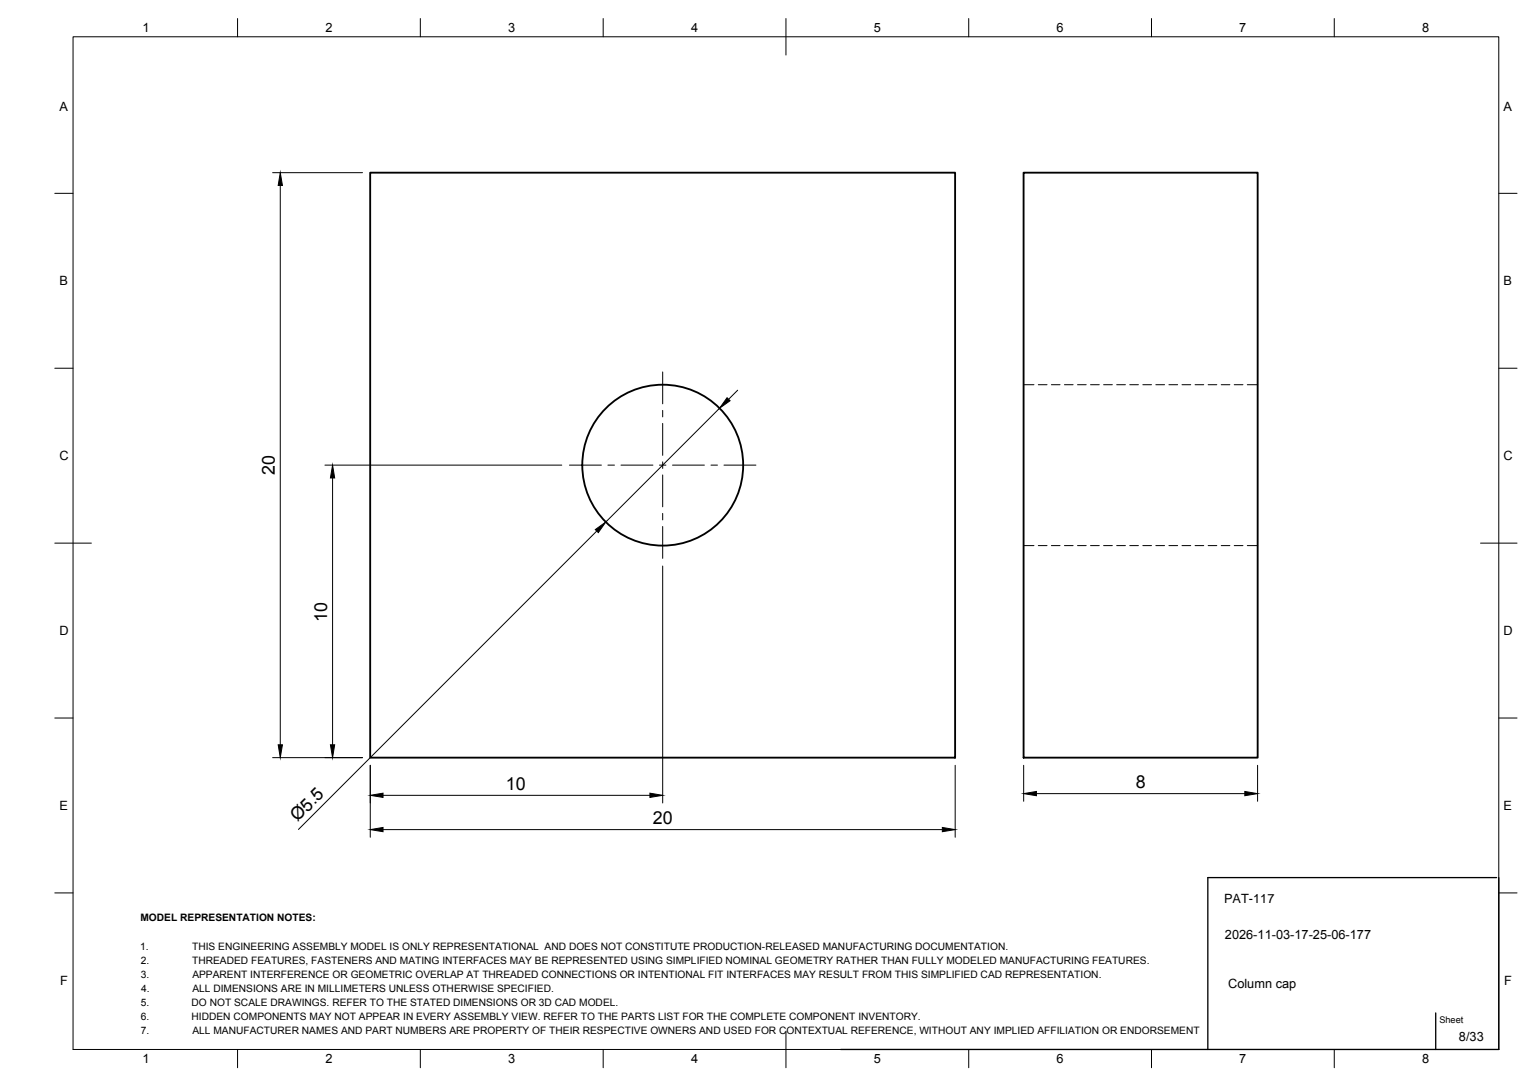
ISO-10303-21;
HEADER;
/* Generated by software containing ST-Developer
 * from STEP Tools, Inc. (www.steptools.com) 
 */

FILE_DESCRIPTION(
/* description */ ('Counterbalanced vertical column'),
/* implementation_level */ '2;1');

FILE_NAME(
/* name */ 'Column cap.step',
/* time_stamp */ '2026-10-29T16:47:22-07:00',
/* author */ (''),
/* organization */ (''),
/* preprocessor_version */ 'ST-DEVELOPER v20.2',
/* originating_system */ 'Autodesk Translation Framework v15.17.0.0',
/* authorisation */ '');

FILE_SCHEMA (('AUTOMOTIVE_DESIGN { 1 0 10303 214 3 1 1 }'));
ENDSEC;

DATA;
#10=MECHANICAL_DESIGN_GEOMETRIC_PRESENTATION_REPRESENTATION('',(#353),#15040);
#283=SHAPE_REPRESENTATION_RELATIONSHIP('SRR','None',#15187,#318);
#318=ADVANCED_BREP_SHAPE_REPRESENTATION('',(#388),#15006);
#353=STYLED_ITEM('',(#15471),#388);
#388=MANIFOLD_SOLID_BREP('Body1',#7076);
#422=FACE_BOUND('',#1270,.T.);
#423=FACE_BOUND('',#1272,.T.);
#553=PLANE('',#7544);
#554=PLANE('',#7545);
#555=PLANE('',#7546);
#556=PLANE('',#7547);
#557=PLANE('',#7548);
#558=PLANE('',#7549);
#853=FACE_OUTER_BOUND('',#1264,.T.);
#854=FACE_OUTER_BOUND('',#1265,.T.);
#855=FACE_OUTER_BOUND('',#1266,.T.);
#856=FACE_OUTER_BOUND('',#1267,.T.);
#857=FACE_OUTER_BOUND('',#1268,.T.);
#858=FACE_OUTER_BOUND('',#1269,.T.);
#859=FACE_OUTER_BOUND('',#1271,.T.);
#1264=EDGE_LOOP('',(#4890,#4891,#4892,#4893));
#1265=EDGE_LOOP('',(#4894,#4895,#4896,#4897));
#1266=EDGE_LOOP('',(#4898,#4899,#4900,#4901));
#1267=EDGE_LOOP('',(#4902,#4903,#4904,#4905));
#1268=EDGE_LOOP('',(#4906,#4907,#4908,#4909));
#1269=EDGE_LOOP('',(#4910,#4911,#4912,#4913));
#1270=EDGE_LOOP('',(#4914));
#1271=EDGE_LOOP('',(#4915,#4916,#4917,#4918));
#1272=EDGE_LOOP('',(#4919));
#1792=LINE('',#10460,#2463);
#1793=LINE('',#10465,#2464);
#1794=LINE('',#10467,#2465);
#1795=LINE('',#10469,#2466);
#1796=LINE('',#10470,#2467);
#1797=LINE('',#10473,#2468);
#1798=LINE('',#10475,#2469);
#1799=LINE('',#10476,#2470);
#1800=LINE('',#10479,#2471);
#1801=LINE('',#10481,#2472);
#1802=LINE('',#10482,#2473);
#1803=LINE('',#10484,#2474);
#1804=LINE('',#10485,#2475);
#2463=VECTOR('',#8352,0.275);
#2464=VECTOR('',#8357,1.);
#2465=VECTOR('',#8358,1.);
#2466=VECTOR('',#8359,1.);
#2467=VECTOR('',#8360,1.);
#2468=VECTOR('',#8363,1.);
#2469=VECTOR('',#8364,1.);
#2470=VECTOR('',#8365,1.);
#2471=VECTOR('',#8368,1.);
#2472=VECTOR('',#8369,1.);
#2473=VECTOR('',#8370,1.);
#2474=VECTOR('',#8373,1.);
#2475=VECTOR('',#8374,1.);
#3103=CIRCLE('',#7542,0.275);
#3104=CIRCLE('',#7543,0.275);
#3340=VERTEX_POINT('',#10457);
#3341=VERTEX_POINT('',#10459);
#3342=VERTEX_POINT('',#10463);
#3343=VERTEX_POINT('',#10464);
#3344=VERTEX_POINT('',#10466);
#3345=VERTEX_POINT('',#10468);
#3346=VERTEX_POINT('',#10472);
#3347=VERTEX_POINT('',#10474);
#3348=VERTEX_POINT('',#10478);
#3349=VERTEX_POINT('',#10480);
#3946=EDGE_CURVE('',#3340,#3340,#3103,.T.);
#3947=EDGE_CURVE('',#3340,#3341,#1792,.T.);
#3948=EDGE_CURVE('',#3341,#3341,#3104,.T.);
#3949=EDGE_CURVE('',#3342,#3343,#1793,.T.);
#3950=EDGE_CURVE('',#3343,#3344,#1794,.T.);
#3951=EDGE_CURVE('',#3345,#3344,#1795,.T.);
#3952=EDGE_CURVE('',#3342,#3345,#1796,.T.);
#3953=EDGE_CURVE('',#3346,#3342,#1797,.T.);
#3954=EDGE_CURVE('',#3347,#3345,#1798,.T.);
#3955=EDGE_CURVE('',#3346,#3347,#1799,.T.);
#3956=EDGE_CURVE('',#3348,#3346,#1800,.T.);
#3957=EDGE_CURVE('',#3349,#3347,#1801,.T.);
#3958=EDGE_CURVE('',#3348,#3349,#1802,.T.);
#3959=EDGE_CURVE('',#3343,#3348,#1803,.T.);
#3960=EDGE_CURVE('',#3344,#3349,#1804,.T.);
#4890=ORIENTED_EDGE('',*,*,#3946,.F.);
#4891=ORIENTED_EDGE('',*,*,#3947,.T.);
#4892=ORIENTED_EDGE('',*,*,#3948,.F.);
#4893=ORIENTED_EDGE('',*,*,#3947,.F.);
#4894=ORIENTED_EDGE('',*,*,#3949,.T.);
#4895=ORIENTED_EDGE('',*,*,#3950,.T.);
#4896=ORIENTED_EDGE('',*,*,#3951,.F.);
#4897=ORIENTED_EDGE('',*,*,#3952,.F.);
#4898=ORIENTED_EDGE('',*,*,#3953,.T.);
#4899=ORIENTED_EDGE('',*,*,#3952,.T.);
#4900=ORIENTED_EDGE('',*,*,#3954,.F.);
#4901=ORIENTED_EDGE('',*,*,#3955,.F.);
#4902=ORIENTED_EDGE('',*,*,#3956,.T.);
#4903=ORIENTED_EDGE('',*,*,#3955,.T.);
#4904=ORIENTED_EDGE('',*,*,#3957,.F.);
#4905=ORIENTED_EDGE('',*,*,#3958,.F.);
#4906=ORIENTED_EDGE('',*,*,#3959,.T.);
#4907=ORIENTED_EDGE('',*,*,#3958,.T.);
#4908=ORIENTED_EDGE('',*,*,#3960,.F.);
#4909=ORIENTED_EDGE('',*,*,#3950,.F.);
#4910=ORIENTED_EDGE('',*,*,#3960,.T.);
#4911=ORIENTED_EDGE('',*,*,#3957,.T.);
#4912=ORIENTED_EDGE('',*,*,#3954,.T.);
#4913=ORIENTED_EDGE('',*,*,#3951,.T.);
#4914=ORIENTED_EDGE('',*,*,#3948,.T.);
#4915=ORIENTED_EDGE('',*,*,#3959,.F.);
#4916=ORIENTED_EDGE('',*,*,#3949,.F.);
#4917=ORIENTED_EDGE('',*,*,#3953,.F.);
#4918=ORIENTED_EDGE('',*,*,#3956,.F.);
#4919=ORIENTED_EDGE('',*,*,#3946,.T.);
#6579=CYLINDRICAL_SURFACE('',#7541,0.275);
#6695=ADVANCED_FACE('',(#853),#6579,.F.);
#6696=ADVANCED_FACE('',(#854),#553,.T.);
#6697=ADVANCED_FACE('',(#855),#554,.T.);
#6698=ADVANCED_FACE('',(#856),#555,.T.);
#6699=ADVANCED_FACE('',(#857),#556,.T.);
#6700=ADVANCED_FACE('',(#858,#422),#557,.T.);
#6701=ADVANCED_FACE('',(#859,#423),#558,.F.);
#7076=CLOSED_SHELL('',(#6695,#6696,#6697,#6698,#6699,#6700,#6701));
#7540=AXIS2_PLACEMENT_3D('',#10455,#8346,#8347);
#7541=AXIS2_PLACEMENT_3D('',#10456,#8348,#8349);
#7542=AXIS2_PLACEMENT_3D('',#10458,#8350,#8351);
#7543=AXIS2_PLACEMENT_3D('',#10461,#8353,#8354);
#7544=AXIS2_PLACEMENT_3D('',#10462,#8355,#8356);
#7545=AXIS2_PLACEMENT_3D('',#10471,#8361,#8362);
#7546=AXIS2_PLACEMENT_3D('',#10477,#8366,#8367);
#7547=AXIS2_PLACEMENT_3D('',#10483,#8371,#8372);
#7548=AXIS2_PLACEMENT_3D('',#10486,#8375,#8376);
#7549=AXIS2_PLACEMENT_3D('',#10487,#8377,#8378);
#8346=DIRECTION('axis',(0.,0.,1.));
#8347=DIRECTION('refdir',(1.,0.,0.));
#8348=DIRECTION('center_axis',(0.,0.,1.));
#8349=DIRECTION('ref_axis',(1.,0.,0.));
#8350=DIRECTION('center_axis',(0.,0.,1.));
#8351=DIRECTION('ref_axis',(1.,0.,0.));
#8352=DIRECTION('',(0.,0.,1.));
#8353=DIRECTION('center_axis',(0.,0.,-1.));
#8354=DIRECTION('ref_axis',(1.,0.,0.));
#8355=DIRECTION('center_axis',(0.,1.,0.));
#8356=DIRECTION('ref_axis',(-1.,0.,0.));
#8357=DIRECTION('',(-1.,0.,0.));
#8358=DIRECTION('',(0.,0.,1.));
#8359=DIRECTION('',(-1.,0.,0.));
#8360=DIRECTION('',(0.,0.,1.));
#8361=DIRECTION('center_axis',(1.,0.,0.));
#8362=DIRECTION('ref_axis',(0.,1.,0.));
#8363=DIRECTION('',(0.,1.,0.));
#8364=DIRECTION('',(0.,1.,0.));
#8365=DIRECTION('',(0.,0.,1.));
#8366=DIRECTION('center_axis',(0.,-1.,0.));
#8367=DIRECTION('ref_axis',(1.,0.,0.));
#8368=DIRECTION('',(1.,0.,0.));
#8369=DIRECTION('',(1.,0.,0.));
#8370=DIRECTION('',(0.,0.,1.));
#8371=DIRECTION('center_axis',(-1.,0.,0.));
#8372=DIRECTION('ref_axis',(0.,-1.,0.));
#8373=DIRECTION('',(0.,-1.,0.));
#8374=DIRECTION('',(0.,-1.,0.));
#8375=DIRECTION('center_axis',(0.,0.,1.));
#8376=DIRECTION('ref_axis',(1.,0.,0.));
#8377=DIRECTION('center_axis',(0.,0.,1.));
#8378=DIRECTION('ref_axis',(1.,0.,0.));
#10455=CARTESIAN_POINT('',(0.,0.,0.));
#10456=CARTESIAN_POINT('Origin',(3.,0.,39.9));
#10457=CARTESIAN_POINT('',(2.725,-3.36777869765522E-17,40.));
#10458=CARTESIAN_POINT('Origin',(3.,0.,40.));
#10459=CARTESIAN_POINT('',(2.725,3.36777869765522E-17,40.8));
#10460=CARTESIAN_POINT('',(2.725,-3.36777869765522E-17,39.9));
#10461=CARTESIAN_POINT('Origin',(3.,0.,40.8));
#10462=CARTESIAN_POINT('Origin',(4.,1.,40.));
#10463=CARTESIAN_POINT('',(4.,1.,40.));
#10464=CARTESIAN_POINT('',(2.,1.,40.));
#10465=CARTESIAN_POINT('',(4.,1.,40.));
#10466=CARTESIAN_POINT('',(2.,1.,40.8));
#10467=CARTESIAN_POINT('',(2.,1.,40.));
#10468=CARTESIAN_POINT('',(4.,1.,40.8));
#10469=CARTESIAN_POINT('',(4.,1.,40.8));
#10470=CARTESIAN_POINT('',(4.,1.,40.));
#10471=CARTESIAN_POINT('Origin',(4.,-1.,40.));
#10472=CARTESIAN_POINT('',(4.,-1.,40.));
#10473=CARTESIAN_POINT('',(4.,-1.,40.));
#10474=CARTESIAN_POINT('',(4.,-1.,40.8));
#10475=CARTESIAN_POINT('',(4.,-1.,40.8));
#10476=CARTESIAN_POINT('',(4.,-1.,40.));
#10477=CARTESIAN_POINT('Origin',(2.,-1.,40.));
#10478=CARTESIAN_POINT('',(2.,-1.,40.));
#10479=CARTESIAN_POINT('',(2.,-1.,40.));
#10480=CARTESIAN_POINT('',(2.,-1.,40.8));
#10481=CARTESIAN_POINT('',(2.,-1.,40.8));
#10482=CARTESIAN_POINT('',(2.,-1.,40.));
#10483=CARTESIAN_POINT('Origin',(2.,1.,40.));
#10484=CARTESIAN_POINT('',(2.,1.,40.));
#10485=CARTESIAN_POINT('',(2.,1.,40.8));
#10486=CARTESIAN_POINT('Origin',(3.,0.,40.8));
#10487=CARTESIAN_POINT('Origin',(3.,0.,40.));
#14966=UNCERTAINTY_MEASURE_WITH_UNIT(LENGTH_MEASURE(0.001),#15041,
'DISTANCE_ACCURACY_VALUE',
'Maximum model space distance between geometric entities at asserted c
onnectivities');
#15000=UNCERTAINTY_MEASURE_WITH_UNIT(LENGTH_MEASURE(0.001),#15041,
'DISTANCE_ACCURACY_VALUE',
'Maximum model space distance between geometric entities at asserted c
onnectivities');
#15006=(
GEOMETRIC_REPRESENTATION_CONTEXT(3)
GLOBAL_UNCERTAINTY_ASSIGNED_CONTEXT((#14966))
GLOBAL_UNIT_ASSIGNED_CONTEXT((#15041,#15043,#15044))
REPRESENTATION_CONTEXT('','3D')
);
#15040=(
GEOMETRIC_REPRESENTATION_CONTEXT(3)
GLOBAL_UNCERTAINTY_ASSIGNED_CONTEXT((#15000))
GLOBAL_UNIT_ASSIGNED_CONTEXT((#15041,#15043,#15044))
REPRESENTATION_CONTEXT('','3D')
);
#15041=(
LENGTH_UNIT()
NAMED_UNIT(*)
SI_UNIT(.CENTI.,.METRE.)
);
#15043=(
NAMED_UNIT(*)
PLANE_ANGLE_UNIT()
SI_UNIT($,.RADIAN.)
);
#15044=(
NAMED_UNIT(*)
SI_UNIT($,.STERADIAN.)
SOLID_ANGLE_UNIT()
);
#15050=SHAPE_DEFINITION_REPRESENTATION(#15089,#15187);
#15089=PRODUCT_DEFINITION_SHAPE('',$,#15227);
#15187=SHAPE_REPRESENTATION('',(#7540),#15006);
#15221=PRODUCT_DEFINITION_CONTEXT('part definition',#15340,'design');
#15227=PRODUCT_DEFINITION('Column cap','Column cap',#15266,#15221);
#15266=PRODUCT_DEFINITION_FORMATION('',$,#15347);
#15340=APPLICATION_CONTEXT(
'Core Data for Automotive Mechanical Design Process');
#15341=PRODUCT_CONTEXT('part definition',#15340,'mechanical');
#15347=PRODUCT('Column cap','Column cap','Column cap',(#15341));
#15465=COLOUR_RGB('Off White',0.89,0.88,0.83);
#15466=FILL_AREA_STYLE_COLOUR('',#15465);
#15467=FILL_AREA_STYLE('',(#15466));
#15468=SURFACE_STYLE_FILL_AREA(#15467);
#15469=SURFACE_SIDE_STYLE('',(#15468));
#15470=SURFACE_STYLE_USAGE(.BOTH.,#15469);
#15471=PRESENTATION_STYLE_ASSIGNMENT((#15470));
ENDSEC;
END-ISO-10303-21;
